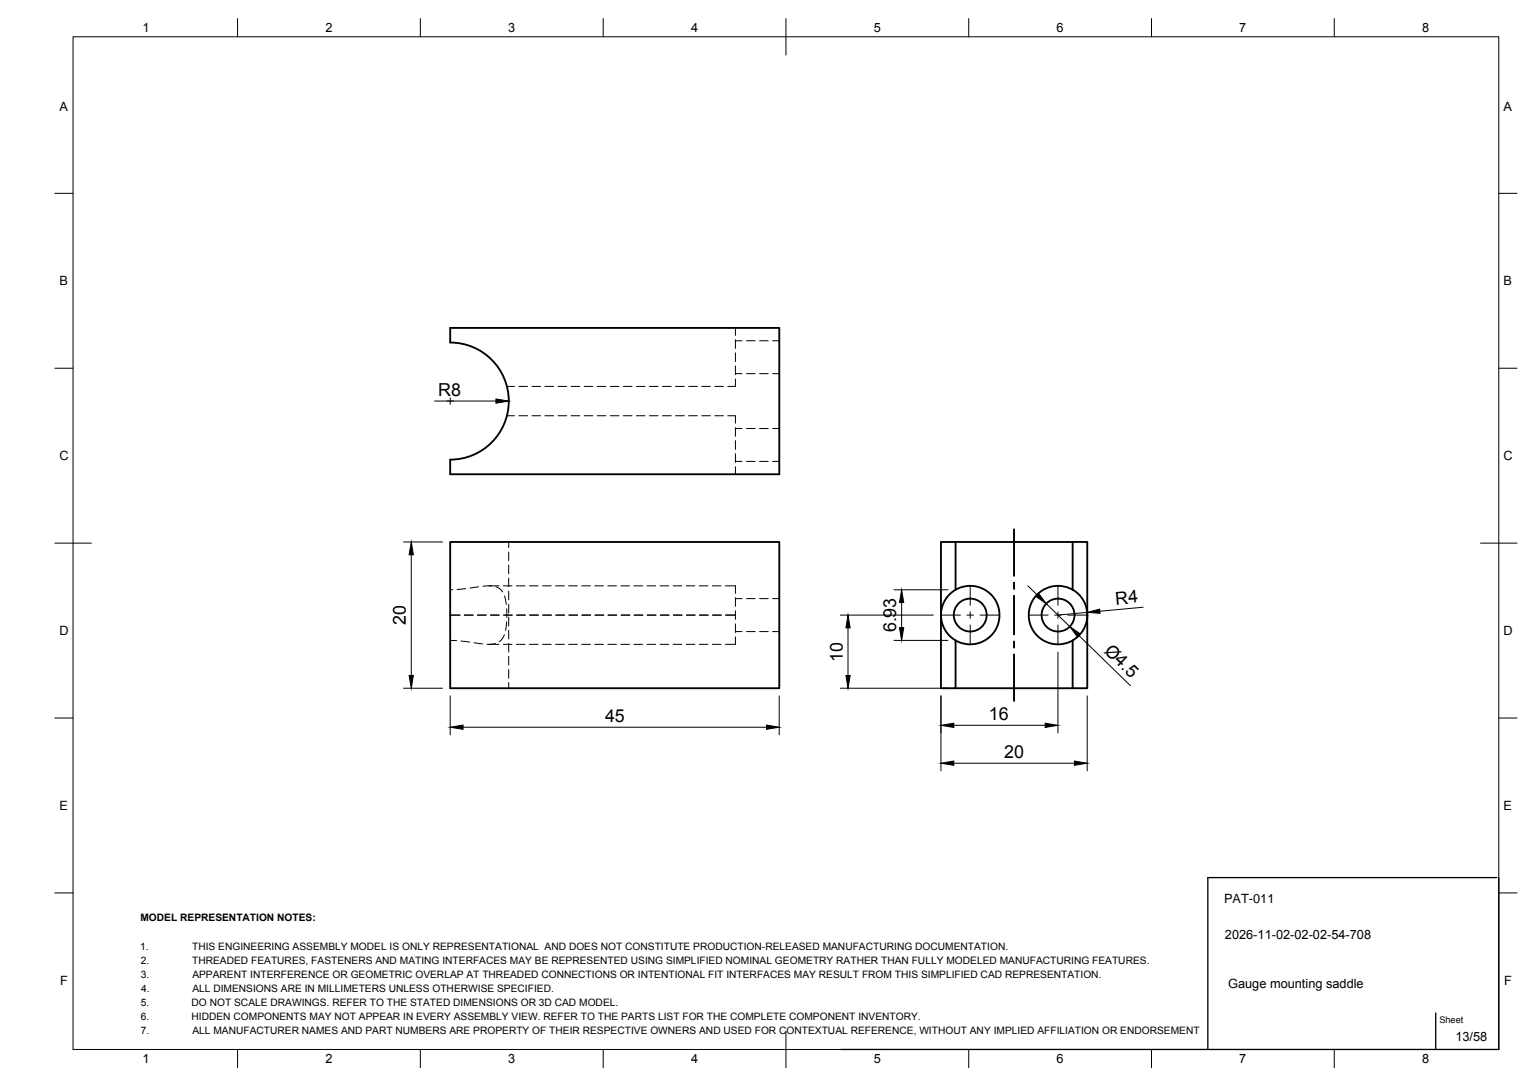
ISO-10303-21;
HEADER;
/* Generated by software containing ST-Developer
 * from STEP Tools, Inc. (www.steptools.com) 
 */

FILE_DESCRIPTION(
/* description */ ('Belt tension measurement rig'),
/* implementation_level */ '2;1');

FILE_NAME(
/* name */ 'Gauge mounting saddle.step',
/* time_stamp */ '2026-10-28T03:24:44-07:00',
/* author */ (''),
/* organization */ (''),
/* preprocessor_version */ 'ST-DEVELOPER v20.2',
/* originating_system */ 'Autodesk Translation Framework v15.17.0.0',
/* authorisation */ '');

FILE_SCHEMA (('AUTOMOTIVE_DESIGN { 1 0 10303 214 3 1 1 }'));
ENDSEC;

DATA;
#10=MECHANICAL_DESIGN_GEOMETRIC_PRESENTATION_REPRESENTATION('',(#704),#23587);
#491=B_SPLINE_CURVE_WITH_KNOTS('',3,(#19153,#19154,#19155,#19156,#19157,
#19158),.UNSPECIFIED.,.F.,.F.,(4,2,4),(1.88587037555333,2.15501811419061,
2.44576925996922),.UNSPECIFIED.);
#492=B_SPLINE_CURVE_WITH_KNOTS('',3,(#19169,#19170,#19171,#19172,#19173,
#19174,#19175,#19176,#19177,#19178,#19179,#19180,#19181,#19182,#19183,#19184,
#19185,#19186,#19187,#19188,#19189,#19190,#19191,#19192,#19193,#19194,#19195,
#19196,#19197,#19198,#19199,#19200),.UNSPECIFIED.,.F.,.F.,(4,2,2,2,2,2,
2,2,2,2,2,2,2,2,2,4),(0.559898884415891,0.581502291557221,0.697930042244281,
0.814357792931341,0.918959320915763,1.02356084890019,1.1232227394424,1.22288462998461,
1.32254652052682,1.42220841106903,1.52680993905346,1.63141146703788,1.74783921772494,
1.864266968412,2.15501811419061,2.44576925996922),.UNSPECIFIED.);
#493=B_SPLINE_CURVE_WITH_KNOTS('',3,(#19203,#19204,#19205,#19206,#19207,
#19208),.UNSPECIFIED.,.F.,.F.,(4,2,4),(0.,0.29075114577861,0.559898884415891),
 .UNSPECIFIED.);
#494=B_SPLINE_CURVE_WITH_KNOTS('',3,(#19217,#19218,#19219,#19220,#19221,
#19222,#19223,#19224,#19225,#19226,#19227,#19228,#19229,#19230,#19231,#19232,
#19233,#19234,#19235,#19236,#19237,#19238,#19239,#19240,#19241,#19242,#19243,
#19244,#19245,#19246,#19247,#19248),.UNSPECIFIED.,.F.,.F.,(4,2,2,2,2,2,
2,2,2,2,2,2,2,2,2,4),(0.,0.29075114577861,0.58150229155722,0.69793004224428,
0.814357792931341,0.918959320915763,1.02356084890019,1.1232227394424,1.22288462998461,
1.32254652052682,1.42220841106904,1.52680993905346,1.63141146703788,1.74783921772494,
1.864266968412,1.88587037555333),.UNSPECIFIED.);
#594=SHAPE_REPRESENTATION_RELATIONSHIP('SRR','None',#23839,#649);
#649=ADVANCED_BREP_SHAPE_REPRESENTATION('',(#774),#23537);
#704=STYLED_ITEM('',(#24197),#774);
#774=MANIFOLD_SOLID_BREP('Body1',#12209);
#891=FACE_BOUND('',#2255,.T.);
#892=FACE_BOUND('',#2258,.T.);
#893=FACE_BOUND('',#2271,.T.);
#894=FACE_BOUND('',#2272,.T.);
#1109=PLANE('',#13155);
#1110=PLANE('',#13160);
#1111=PLANE('',#13162);
#1112=PLANE('',#13163);
#1113=PLANE('',#13164);
#1114=PLANE('',#13172);
#1115=PLANE('',#13173);
#1116=PLANE('',#13174);
#1117=PLANE('',#13175);
#1118=PLANE('',#13176);
#1119=PLANE('',#13177);
#1485=FACE_OUTER_BOUND('',#2251,.T.);
#1486=FACE_OUTER_BOUND('',#2252,.T.);
#1487=FACE_OUTER_BOUND('',#2253,.T.);
#1488=FACE_OUTER_BOUND('',#2254,.T.);
#1489=FACE_OUTER_BOUND('',#2256,.T.);
#1490=FACE_OUTER_BOUND('',#2257,.T.);
#1491=FACE_OUTER_BOUND('',#2259,.T.);
#1492=FACE_OUTER_BOUND('',#2260,.T.);
#1493=FACE_OUTER_BOUND('',#2261,.T.);
#1494=FACE_OUTER_BOUND('',#2262,.T.);
#1495=FACE_OUTER_BOUND('',#2263,.T.);
#1496=FACE_OUTER_BOUND('',#2264,.T.);
#1497=FACE_OUTER_BOUND('',#2265,.T.);
#1498=FACE_OUTER_BOUND('',#2266,.T.);
#1499=FACE_OUTER_BOUND('',#2267,.T.);
#1500=FACE_OUTER_BOUND('',#2268,.T.);
#1501=FACE_OUTER_BOUND('',#2269,.T.);
#1502=FACE_OUTER_BOUND('',#2270,.T.);
#2251=EDGE_LOOP('',(#8472,#8473,#8474,#8475,#8476));
#2252=EDGE_LOOP('',(#8477,#8478,#8479,#8480,#8481));
#2253=EDGE_LOOP('',(#8482,#8483,#8484,#8485,#8486));
#2254=EDGE_LOOP('',(#8487,#8488));
#2255=EDGE_LOOP('',(#8489));
#2256=EDGE_LOOP('',(#8490,#8491,#8492,#8493,#8494));
#2257=EDGE_LOOP('',(#8495,#8496));
#2258=EDGE_LOOP('',(#8497));
#2259=EDGE_LOOP('',(#8498,#8499,#8500,#8501));
#2260=EDGE_LOOP('',(#8502,#8503,#8504,#8505));
#2261=EDGE_LOOP('',(#8506,#8507,#8508,#8509));
#2262=EDGE_LOOP('',(#8510,#8511,#8512,#8513));
#2263=EDGE_LOOP('',(#8514,#8515,#8516,#8517));
#2264=EDGE_LOOP('',(#8518,#8519,#8520,#8521,#8522,#8523,#8524,#8525,#8526,
#8527));
#2265=EDGE_LOOP('',(#8528,#8529,#8530,#8531,#8532,#8533));
#2266=EDGE_LOOP('',(#8534,#8535,#8536,#8537));
#2267=EDGE_LOOP('',(#8538,#8539,#8540,#8541,#8542,#8543,#8544));
#2268=EDGE_LOOP('',(#8545,#8546,#8547,#8548,#8549,#8550,#8551));
#2269=EDGE_LOOP('',(#8552,#8553,#8554,#8555,#8556,#8557));
#2270=EDGE_LOOP('',(#8558,#8559,#8560,#8561));
#2271=EDGE_LOOP('',(#8562));
#2272=EDGE_LOOP('',(#8563));
#3113=LINE('',#19146,#3864);
#3114=LINE('',#19150,#3865);
#3115=LINE('',#19162,#3866);
#3116=LINE('',#19166,#3867);
#3117=LINE('',#19210,#3868);
#3118=LINE('',#19250,#3869);
#3119=LINE('',#19257,#3870);
#3120=LINE('',#19259,#3871);
#3121=LINE('',#19260,#3872);
#3122=LINE('',#19263,#3873);
#3123=LINE('',#19265,#3874);
#3124=LINE('',#19266,#3875);
#3125=LINE('',#19269,#3876);
#3126=LINE('',#19271,#3877);
#3127=LINE('',#19272,#3878);
#3128=LINE('',#19276,#3879);
#3129=LINE('',#19280,#3880);
#3130=LINE('',#19283,#3881);
#3131=LINE('',#19288,#3882);
#3132=LINE('',#19290,#3883);
#3133=LINE('',#19292,#3884);
#3134=LINE('',#19293,#3885);
#3135=LINE('',#19295,#3886);
#3136=LINE('',#19298,#3887);
#3137=LINE('',#19299,#3888);
#3138=LINE('',#19302,#3889);
#3139=LINE('',#19303,#3890);
#3140=LINE('',#19305,#3891);
#3864=VECTOR('',#15204,0.4);
#3865=VECTOR('',#15207,1.);
#3866=VECTOR('',#15212,0.4);
#3867=VECTOR('',#15215,1.);
#3868=VECTOR('',#15222,1.);
#3869=VECTOR('',#15233,1.);
#3870=VECTOR('',#15242,1.);
#3871=VECTOR('',#15243,1.);
#3872=VECTOR('',#15244,1.);
#3873=VECTOR('',#15247,1.);
#3874=VECTOR('',#15248,1.);
#3875=VECTOR('',#15249,1.);
#3876=VECTOR('',#15252,1.);
#3877=VECTOR('',#15253,1.);
#3878=VECTOR('',#15254,1.);
#3879=VECTOR('',#15259,0.225);
#3880=VECTOR('',#15264,0.225);
#3881=VECTOR('',#15267,1.);
#3882=VECTOR('',#15274,1.);
#3883=VECTOR('',#15275,1.);
#3884=VECTOR('',#15276,1.);
#3885=VECTOR('',#15277,1.);
#3886=VECTOR('',#15280,1.);
#3887=VECTOR('',#15283,1.);
#3888=VECTOR('',#15284,1.);
#3889=VECTOR('',#15287,1.);
#3890=VECTOR('',#15288,1.);
#3891=VECTOR('',#15291,1.);
#4592=CIRCLE('',#13147,0.4);
#4593=CIRCLE('',#13148,0.4);
#4594=CIRCLE('',#13150,0.4);
#4595=CIRCLE('',#13151,0.4);
#4596=CIRCLE('',#13153,0.4);
#4597=CIRCLE('',#13154,0.4);
#4598=CIRCLE('',#13156,0.225);
#4599=CIRCLE('',#13158,0.4);
#4600=CIRCLE('',#13159,0.4);
#4601=CIRCLE('',#13161,0.225);
#4602=CIRCLE('',#13166,0.225);
#4603=CIRCLE('',#13168,0.225);
#4604=CIRCLE('',#13170,0.8);
#4605=CIRCLE('',#13171,0.8);
#5416=VERTEX_POINT('',#19144);
#5417=VERTEX_POINT('',#19145);
#5418=VERTEX_POINT('',#19147);
#5419=VERTEX_POINT('',#19149);
#5420=VERTEX_POINT('',#19151);
#5421=VERTEX_POINT('',#19160);
#5422=VERTEX_POINT('',#19161);
#5423=VERTEX_POINT('',#19163);
#5424=VERTEX_POINT('',#19165);
#5425=VERTEX_POINT('',#19167);
#5426=VERTEX_POINT('',#19202);
#5427=VERTEX_POINT('',#19213);
#5428=VERTEX_POINT('',#19216);
#5429=VERTEX_POINT('',#19253);
#5430=VERTEX_POINT('',#19256);
#5431=VERTEX_POINT('',#19258);
#5432=VERTEX_POINT('',#19262);
#5433=VERTEX_POINT('',#19264);
#5434=VERTEX_POINT('',#19268);
#5435=VERTEX_POINT('',#19270);
#5436=VERTEX_POINT('',#19274);
#5437=VERTEX_POINT('',#19278);
#5438=VERTEX_POINT('',#19282);
#5439=VERTEX_POINT('',#19287);
#5440=VERTEX_POINT('',#19289);
#5441=VERTEX_POINT('',#19291);
#5442=VERTEX_POINT('',#19297);
#5443=VERTEX_POINT('',#19301);
#6595=EDGE_CURVE('',#5416,#5417,#3113,.T.);
#6596=EDGE_CURVE('',#5418,#5416,#4592,.T.);
#6597=EDGE_CURVE('',#5418,#5419,#3114,.T.);
#6598=EDGE_CURVE('',#5420,#5419,#4593,.T.);
#6599=EDGE_CURVE('',#5417,#5420,#491,.T.);
#6600=EDGE_CURVE('',#5421,#5422,#3115,.T.);
#6601=EDGE_CURVE('',#5423,#5421,#4594,.T.);
#6602=EDGE_CURVE('',#5423,#5424,#3116,.T.);
#6603=EDGE_CURVE('',#5425,#5424,#4595,.T.);
#6604=EDGE_CURVE('',#5422,#5425,#492,.T.);
#6605=EDGE_CURVE('',#5426,#5422,#493,.T.);
#6606=EDGE_CURVE('',#5424,#5426,#4596,.T.);
#6607=EDGE_CURVE('',#5423,#5424,#3117,.T.);
#6608=EDGE_CURVE('',#5421,#5423,#4597,.T.);
#6609=EDGE_CURVE('',#5427,#5427,#4598,.T.);
#6610=EDGE_CURVE('',#5428,#5417,#494,.T.);
#6611=EDGE_CURVE('',#5419,#5428,#4599,.T.);
#6612=EDGE_CURVE('',#5418,#5419,#3118,.T.);
#6613=EDGE_CURVE('',#5416,#5418,#4600,.T.);
#6614=EDGE_CURVE('',#5429,#5429,#4601,.T.);
#6615=EDGE_CURVE('',#5426,#5430,#3119,.T.);
#6616=EDGE_CURVE('',#5430,#5431,#3120,.T.);
#6617=EDGE_CURVE('',#5431,#5424,#3121,.T.);
#6618=EDGE_CURVE('',#5428,#5432,#3122,.T.);
#6619=EDGE_CURVE('',#5432,#5433,#3123,.T.);
#6620=EDGE_CURVE('',#5433,#5419,#3124,.T.);
#6621=EDGE_CURVE('',#5419,#5434,#3125,.T.);
#6622=EDGE_CURVE('',#5434,#5435,#3126,.T.);
#6623=EDGE_CURVE('',#5435,#5420,#3127,.T.);
#6624=EDGE_CURVE('',#5436,#5436,#4602,.T.);
#6625=EDGE_CURVE('',#5436,#5427,#3128,.T.);
#6626=EDGE_CURVE('',#5437,#5437,#4603,.T.);
#6627=EDGE_CURVE('',#5437,#5429,#3129,.T.);
#6628=EDGE_CURVE('',#5438,#5425,#3130,.T.);
#6629=EDGE_CURVE('',#5432,#5438,#4604,.T.);
#6630=EDGE_CURVE('',#5430,#5435,#4605,.T.);
#6631=EDGE_CURVE('',#5439,#5438,#3131,.T.);
#6632=EDGE_CURVE('',#5440,#5439,#3132,.T.);
#6633=EDGE_CURVE('',#5440,#5441,#3133,.T.);
#6634=EDGE_CURVE('',#5441,#5433,#3134,.T.);
#6635=EDGE_CURVE('',#5424,#5439,#3135,.T.);
#6636=EDGE_CURVE('',#5441,#5442,#3136,.T.);
#6637=EDGE_CURVE('',#5442,#5434,#3137,.T.);
#6638=EDGE_CURVE('',#5443,#5440,#3138,.T.);
#6639=EDGE_CURVE('',#5443,#5431,#3139,.T.);
#6640=EDGE_CURVE('',#5442,#5443,#3140,.T.);
#8472=ORIENTED_EDGE('',*,*,#6595,.F.);
#8473=ORIENTED_EDGE('',*,*,#6596,.F.);
#8474=ORIENTED_EDGE('',*,*,#6597,.T.);
#8475=ORIENTED_EDGE('',*,*,#6598,.F.);
#8476=ORIENTED_EDGE('',*,*,#6599,.F.);
#8477=ORIENTED_EDGE('',*,*,#6600,.F.);
#8478=ORIENTED_EDGE('',*,*,#6601,.F.);
#8479=ORIENTED_EDGE('',*,*,#6602,.T.);
#8480=ORIENTED_EDGE('',*,*,#6603,.F.);
#8481=ORIENTED_EDGE('',*,*,#6604,.F.);
#8482=ORIENTED_EDGE('',*,*,#6600,.T.);
#8483=ORIENTED_EDGE('',*,*,#6605,.F.);
#8484=ORIENTED_EDGE('',*,*,#6606,.F.);
#8485=ORIENTED_EDGE('',*,*,#6607,.F.);
#8486=ORIENTED_EDGE('',*,*,#6608,.F.);
#8487=ORIENTED_EDGE('',*,*,#6601,.T.);
#8488=ORIENTED_EDGE('',*,*,#6608,.T.);
#8489=ORIENTED_EDGE('',*,*,#6609,.F.);
#8490=ORIENTED_EDGE('',*,*,#6595,.T.);
#8491=ORIENTED_EDGE('',*,*,#6610,.F.);
#8492=ORIENTED_EDGE('',*,*,#6611,.F.);
#8493=ORIENTED_EDGE('',*,*,#6612,.F.);
#8494=ORIENTED_EDGE('',*,*,#6613,.F.);
#8495=ORIENTED_EDGE('',*,*,#6596,.T.);
#8496=ORIENTED_EDGE('',*,*,#6613,.T.);
#8497=ORIENTED_EDGE('',*,*,#6614,.F.);
#8498=ORIENTED_EDGE('',*,*,#6606,.T.);
#8499=ORIENTED_EDGE('',*,*,#6615,.T.);
#8500=ORIENTED_EDGE('',*,*,#6616,.T.);
#8501=ORIENTED_EDGE('',*,*,#6617,.T.);
#8502=ORIENTED_EDGE('',*,*,#6611,.T.);
#8503=ORIENTED_EDGE('',*,*,#6618,.T.);
#8504=ORIENTED_EDGE('',*,*,#6619,.T.);
#8505=ORIENTED_EDGE('',*,*,#6620,.T.);
#8506=ORIENTED_EDGE('',*,*,#6598,.T.);
#8507=ORIENTED_EDGE('',*,*,#6621,.T.);
#8508=ORIENTED_EDGE('',*,*,#6622,.T.);
#8509=ORIENTED_EDGE('',*,*,#6623,.T.);
#8510=ORIENTED_EDGE('',*,*,#6624,.F.);
#8511=ORIENTED_EDGE('',*,*,#6625,.T.);
#8512=ORIENTED_EDGE('',*,*,#6609,.T.);
#8513=ORIENTED_EDGE('',*,*,#6625,.F.);
#8514=ORIENTED_EDGE('',*,*,#6626,.F.);
#8515=ORIENTED_EDGE('',*,*,#6627,.T.);
#8516=ORIENTED_EDGE('',*,*,#6614,.T.);
#8517=ORIENTED_EDGE('',*,*,#6627,.F.);
#8518=ORIENTED_EDGE('',*,*,#6605,.T.);
#8519=ORIENTED_EDGE('',*,*,#6604,.T.);
#8520=ORIENTED_EDGE('',*,*,#6628,.F.);
#8521=ORIENTED_EDGE('',*,*,#6629,.F.);
#8522=ORIENTED_EDGE('',*,*,#6618,.F.);
#8523=ORIENTED_EDGE('',*,*,#6610,.T.);
#8524=ORIENTED_EDGE('',*,*,#6599,.T.);
#8525=ORIENTED_EDGE('',*,*,#6623,.F.);
#8526=ORIENTED_EDGE('',*,*,#6630,.F.);
#8527=ORIENTED_EDGE('',*,*,#6615,.F.);
#8528=ORIENTED_EDGE('',*,*,#6629,.T.);
#8529=ORIENTED_EDGE('',*,*,#6631,.F.);
#8530=ORIENTED_EDGE('',*,*,#6632,.F.);
#8531=ORIENTED_EDGE('',*,*,#6633,.T.);
#8532=ORIENTED_EDGE('',*,*,#6634,.T.);
#8533=ORIENTED_EDGE('',*,*,#6619,.F.);
#8534=ORIENTED_EDGE('',*,*,#6603,.T.);
#8535=ORIENTED_EDGE('',*,*,#6635,.T.);
#8536=ORIENTED_EDGE('',*,*,#6631,.T.);
#8537=ORIENTED_EDGE('',*,*,#6628,.T.);
#8538=ORIENTED_EDGE('',*,*,#6636,.T.);
#8539=ORIENTED_EDGE('',*,*,#6637,.T.);
#8540=ORIENTED_EDGE('',*,*,#6621,.F.);
#8541=ORIENTED_EDGE('',*,*,#6597,.F.);
#8542=ORIENTED_EDGE('',*,*,#6612,.T.);
#8543=ORIENTED_EDGE('',*,*,#6620,.F.);
#8544=ORIENTED_EDGE('',*,*,#6634,.F.);
#8545=ORIENTED_EDGE('',*,*,#6638,.T.);
#8546=ORIENTED_EDGE('',*,*,#6632,.T.);
#8547=ORIENTED_EDGE('',*,*,#6635,.F.);
#8548=ORIENTED_EDGE('',*,*,#6602,.F.);
#8549=ORIENTED_EDGE('',*,*,#6607,.T.);
#8550=ORIENTED_EDGE('',*,*,#6617,.F.);
#8551=ORIENTED_EDGE('',*,*,#6639,.F.);
#8552=ORIENTED_EDGE('',*,*,#6630,.T.);
#8553=ORIENTED_EDGE('',*,*,#6622,.F.);
#8554=ORIENTED_EDGE('',*,*,#6637,.F.);
#8555=ORIENTED_EDGE('',*,*,#6640,.T.);
#8556=ORIENTED_EDGE('',*,*,#6639,.T.);
#8557=ORIENTED_EDGE('',*,*,#6616,.F.);
#8558=ORIENTED_EDGE('',*,*,#6640,.F.);
#8559=ORIENTED_EDGE('',*,*,#6636,.F.);
#8560=ORIENTED_EDGE('',*,*,#6633,.F.);
#8561=ORIENTED_EDGE('',*,*,#6638,.F.);
#8562=ORIENTED_EDGE('',*,*,#6624,.T.);
#8563=ORIENTED_EDGE('',*,*,#6626,.T.);
#11219=CYLINDRICAL_SURFACE('',#13146,0.4);
#11220=CYLINDRICAL_SURFACE('',#13149,0.4);
#11221=CYLINDRICAL_SURFACE('',#13152,0.4);
#11222=CYLINDRICAL_SURFACE('',#13157,0.4);
#11223=CYLINDRICAL_SURFACE('',#13165,0.225);
#11224=CYLINDRICAL_SURFACE('',#13167,0.225);
#11225=CYLINDRICAL_SURFACE('',#13169,0.8);
#11626=ADVANCED_FACE('',(#1485),#11219,.F.);
#11627=ADVANCED_FACE('',(#1486),#11220,.F.);
#11628=ADVANCED_FACE('',(#1487),#11221,.F.);
#11629=ADVANCED_FACE('',(#1488,#891),#1109,.T.);
#11630=ADVANCED_FACE('',(#1489),#11222,.F.);
#11631=ADVANCED_FACE('',(#1490,#892),#1110,.T.);
#11632=ADVANCED_FACE('',(#1491),#1111,.T.);
#11633=ADVANCED_FACE('',(#1492),#1112,.T.);
#11634=ADVANCED_FACE('',(#1493),#1113,.T.);
#11635=ADVANCED_FACE('',(#1494),#11223,.F.);
#11636=ADVANCED_FACE('',(#1495),#11224,.F.);
#11637=ADVANCED_FACE('',(#1496),#11225,.F.);
#11638=ADVANCED_FACE('',(#1497),#1114,.T.);
#11639=ADVANCED_FACE('',(#1498),#1115,.T.);
#11640=ADVANCED_FACE('',(#1499),#1116,.T.);
#11641=ADVANCED_FACE('',(#1500),#1117,.T.);
#11642=ADVANCED_FACE('',(#1501),#1118,.T.);
#11643=ADVANCED_FACE('',(#1502,#893,#894),#1119,.F.);
#12209=CLOSED_SHELL('',(#11626,#11627,#11628,#11629,#11630,#11631,#11632,
#11633,#11634,#11635,#11636,#11637,#11638,#11639,#11640,#11641,#11642,#11643));
#13145=AXIS2_PLACEMENT_3D('',#19142,#15200,#15201);
#13146=AXIS2_PLACEMENT_3D('',#19143,#15202,#15203);
#13147=AXIS2_PLACEMENT_3D('',#19148,#15205,#15206);
#13148=AXIS2_PLACEMENT_3D('',#19152,#15208,#15209);
#13149=AXIS2_PLACEMENT_3D('',#19159,#15210,#15211);
#13150=AXIS2_PLACEMENT_3D('',#19164,#15213,#15214);
#13151=AXIS2_PLACEMENT_3D('',#19168,#15216,#15217);
#13152=AXIS2_PLACEMENT_3D('',#19201,#15218,#15219);
#13153=AXIS2_PLACEMENT_3D('',#19209,#15220,#15221);
#13154=AXIS2_PLACEMENT_3D('',#19211,#15223,#15224);
#13155=AXIS2_PLACEMENT_3D('',#19212,#15225,#15226);
#13156=AXIS2_PLACEMENT_3D('',#19214,#15227,#15228);
#13157=AXIS2_PLACEMENT_3D('',#19215,#15229,#15230);
#13158=AXIS2_PLACEMENT_3D('',#19249,#15231,#15232);
#13159=AXIS2_PLACEMENT_3D('',#19251,#15234,#15235);
#13160=AXIS2_PLACEMENT_3D('',#19252,#15236,#15237);
#13161=AXIS2_PLACEMENT_3D('',#19254,#15238,#15239);
#13162=AXIS2_PLACEMENT_3D('',#19255,#15240,#15241);
#13163=AXIS2_PLACEMENT_3D('',#19261,#15245,#15246);
#13164=AXIS2_PLACEMENT_3D('',#19267,#15250,#15251);
#13165=AXIS2_PLACEMENT_3D('',#19273,#15255,#15256);
#13166=AXIS2_PLACEMENT_3D('',#19275,#15257,#15258);
#13167=AXIS2_PLACEMENT_3D('',#19277,#15260,#15261);
#13168=AXIS2_PLACEMENT_3D('',#19279,#15262,#15263);
#13169=AXIS2_PLACEMENT_3D('',#19281,#15265,#15266);
#13170=AXIS2_PLACEMENT_3D('',#19284,#15268,#15269);
#13171=AXIS2_PLACEMENT_3D('',#19285,#15270,#15271);
#13172=AXIS2_PLACEMENT_3D('',#19286,#15272,#15273);
#13173=AXIS2_PLACEMENT_3D('',#19294,#15278,#15279);
#13174=AXIS2_PLACEMENT_3D('',#19296,#15281,#15282);
#13175=AXIS2_PLACEMENT_3D('',#19300,#15285,#15286);
#13176=AXIS2_PLACEMENT_3D('',#19304,#15289,#15290);
#13177=AXIS2_PLACEMENT_3D('',#19306,#15292,#15293);
#15200=DIRECTION('axis',(0.,0.,1.));
#15201=DIRECTION('refdir',(1.,0.,0.));
#15202=DIRECTION('center_axis',(0.,0.,1.));
#15203=DIRECTION('ref_axis',(1.,0.,0.));
#15204=DIRECTION('',(0.,0.,1.));
#15205=DIRECTION('center_axis',(0.,0.,1.));
#15206=DIRECTION('ref_axis',(1.,0.,0.));
#15207=DIRECTION('',(0.,0.,1.));
#15208=DIRECTION('center_axis',(0.,0.,-1.));
#15209=DIRECTION('ref_axis',(1.,0.,0.));
#15210=DIRECTION('center_axis',(0.,0.,1.));
#15211=DIRECTION('ref_axis',(1.,0.,0.));
#15212=DIRECTION('',(0.,0.,1.));
#15213=DIRECTION('center_axis',(0.,0.,1.));
#15214=DIRECTION('ref_axis',(1.,0.,0.));
#15215=DIRECTION('',(0.,0.,1.));
#15216=DIRECTION('center_axis',(0.,0.,-1.));
#15217=DIRECTION('ref_axis',(1.,0.,0.));
#15218=DIRECTION('center_axis',(0.,0.,1.));
#15219=DIRECTION('ref_axis',(1.,0.,0.));
#15220=DIRECTION('center_axis',(0.,0.,-1.));
#15221=DIRECTION('ref_axis',(1.,0.,0.));
#15222=DIRECTION('',(0.,0.,1.));
#15223=DIRECTION('center_axis',(0.,0.,1.));
#15224=DIRECTION('ref_axis',(1.,0.,0.));
#15225=DIRECTION('center_axis',(0.,0.,1.));
#15226=DIRECTION('ref_axis',(1.,0.,0.));
#15227=DIRECTION('center_axis',(0.,0.,1.));
#15228=DIRECTION('ref_axis',(1.,0.,0.));
#15229=DIRECTION('center_axis',(0.,0.,1.));
#15230=DIRECTION('ref_axis',(1.,0.,0.));
#15231=DIRECTION('center_axis',(0.,0.,-1.));
#15232=DIRECTION('ref_axis',(1.,0.,0.));
#15233=DIRECTION('',(0.,0.,1.));
#15234=DIRECTION('center_axis',(0.,0.,1.));
#15235=DIRECTION('ref_axis',(1.,0.,0.));
#15236=DIRECTION('center_axis',(0.,0.,1.));
#15237=DIRECTION('ref_axis',(1.,0.,0.));
#15238=DIRECTION('center_axis',(0.,0.,1.));
#15239=DIRECTION('ref_axis',(1.,0.,0.));
#15240=DIRECTION('center_axis',(0.,0.,1.));
#15241=DIRECTION('ref_axis',(1.,0.,0.));
#15242=DIRECTION('',(-1.,0.,0.));
#15243=DIRECTION('',(0.,-1.,0.));
#15244=DIRECTION('',(1.,0.,0.));
#15245=DIRECTION('center_axis',(0.,0.,1.));
#15246=DIRECTION('ref_axis',(1.,0.,0.));
#15247=DIRECTION('',(1.,0.,0.));
#15248=DIRECTION('',(0.,1.,0.));
#15249=DIRECTION('',(-1.,0.,0.));
#15250=DIRECTION('center_axis',(0.,0.,1.));
#15251=DIRECTION('ref_axis',(1.,0.,0.));
#15252=DIRECTION('',(-1.,0.,0.));
#15253=DIRECTION('',(0.,-1.,0.));
#15254=DIRECTION('',(1.,0.,0.));
#15255=DIRECTION('center_axis',(0.,0.,1.));
#15256=DIRECTION('ref_axis',(1.,0.,0.));
#15257=DIRECTION('center_axis',(0.,0.,1.));
#15258=DIRECTION('ref_axis',(1.,0.,0.));
#15259=DIRECTION('',(0.,0.,1.));
#15260=DIRECTION('center_axis',(0.,0.,1.));
#15261=DIRECTION('ref_axis',(1.,0.,0.));
#15262=DIRECTION('center_axis',(0.,0.,1.));
#15263=DIRECTION('ref_axis',(1.,0.,0.));
#15264=DIRECTION('',(0.,0.,1.));
#15265=DIRECTION('center_axis',(1.,0.,0.));
#15266=DIRECTION('ref_axis',(0.,0.,-1.));
#15267=DIRECTION('',(-1.,0.,0.));
#15268=DIRECTION('center_axis',(-1.,0.,0.));
#15269=DIRECTION('ref_axis',(0.,0.,-1.));
#15270=DIRECTION('center_axis',(1.,0.,0.));
#15271=DIRECTION('ref_axis',(0.,0.,-1.));
#15272=DIRECTION('center_axis',(1.,0.,0.));
#15273=DIRECTION('ref_axis',(0.,1.,0.));
#15274=DIRECTION('',(0.,1.,0.));
#15275=DIRECTION('',(0.,0.,1.));
#15276=DIRECTION('',(0.,1.,0.));
#15277=DIRECTION('',(0.,0.,1.));
#15278=DIRECTION('center_axis',(0.,0.,1.));
#15279=DIRECTION('ref_axis',(1.,0.,0.));
#15280=DIRECTION('',(1.,0.,0.));
#15281=DIRECTION('center_axis',(0.,1.,0.));
#15282=DIRECTION('ref_axis',(-1.,0.,0.));
#15283=DIRECTION('',(-1.,0.,0.));
#15284=DIRECTION('',(0.,0.,1.));
#15285=DIRECTION('center_axis',(0.,-1.,0.));
#15286=DIRECTION('ref_axis',(1.,0.,0.));
#15287=DIRECTION('',(1.,0.,0.));
#15288=DIRECTION('',(0.,0.,1.));
#15289=DIRECTION('center_axis',(-1.,0.,0.));
#15290=DIRECTION('ref_axis',(0.,-1.,0.));
#15291=DIRECTION('',(0.,-1.,0.));
#15292=DIRECTION('center_axis',(0.,0.,1.));
#15293=DIRECTION('ref_axis',(1.,0.,0.));
#19142=CARTESIAN_POINT('',(0.,0.,0.));
#19143=CARTESIAN_POINT('Origin',(3.,8.1,0.6));
#19144=CARTESIAN_POINT('',(2.6,8.1,0.6));
#19145=CARTESIAN_POINT('',(2.6,8.09999999996984,3.97084973771869));
#19146=CARTESIAN_POINT('',(2.6,8.1,0.6));
#19147=CARTESIAN_POINT('',(3.,8.5,0.6));
#19148=CARTESIAN_POINT('Origin',(3.,8.1,0.6));
#19149=CARTESIAN_POINT('',(3.,8.5,4.5));
#19150=CARTESIAN_POINT('',(3.,8.5,0.6));
#19151=CARTESIAN_POINT('',(2.65358983848623,8.3,4.5));
#19152=CARTESIAN_POINT('Origin',(3.,8.1,4.5));
#19153=CARTESIAN_POINT('Ctrl Pts',(2.6,8.09999999993968,3.97084973771869));
#19154=CARTESIAN_POINT('Ctrl Pts',(2.59999999999099,8.15972702790978,4.0385738216565));
#19155=CARTESIAN_POINT('Ctrl Pts',(2.61364657269785,8.209952841357,4.11951904386589));
#19156=CARTESIAN_POINT('Ctrl Pts',(2.64131535047873,8.28146961928914,4.3010711770996));
#19157=CARTESIAN_POINT('Ctrl Pts',(2.65358983848622,8.3,4.40308295140713));
#19158=CARTESIAN_POINT('Ctrl Pts',(2.65358983848622,8.3,4.5));
#19159=CARTESIAN_POINT('Origin',(3.,6.9,0.6));
#19160=CARTESIAN_POINT('',(2.6,6.9,0.6));
#19161=CARTESIAN_POINT('',(2.6,6.90000000003016,3.97084973771869));
#19162=CARTESIAN_POINT('',(2.6,6.9,0.6));
#19163=CARTESIAN_POINT('',(3.,6.5,0.6));
#19164=CARTESIAN_POINT('Origin',(3.,6.9,0.6));
#19165=CARTESIAN_POINT('',(3.,6.5,4.5));
#19166=CARTESIAN_POINT('',(3.,6.5,0.6));
#19167=CARTESIAN_POINT('',(3.34641016151378,6.7,4.5));
#19168=CARTESIAN_POINT('Origin',(3.,6.9,4.5));
#19169=CARTESIAN_POINT('Ctrl Pts',(2.6,6.90000000006032,3.97084973771869));
#19170=CARTESIAN_POINT('Ctrl Pts',(2.60000000000072,6.90479404852274,3.96541379771789));
#19171=CARTESIAN_POINT('Ctrl Pts',(2.60008620085532,6.90964651743076,3.96006056814498));
#19172=CARTESIAN_POINT('Ctrl Pts',(2.60122740656895,6.94099338970816,3.92640010376094));
#19173=CARTESIAN_POINT('Ctrl Pts',(2.60512454705338,6.97203740815281,3.89755171629685));
#19174=CARTESIAN_POINT('Ctrl Pts',(2.6225443141011,7.03654018405112,3.8466291847403));
#19175=CARTESIAN_POINT('Ctrl Pts',(2.63623381415265,7.06993848403684,3.82453570130603));
#19176=CARTESIAN_POINT('Ctrl Pts',(2.66918291362779,7.12700799839143,3.79158660183088));
#19177=CARTESIAN_POINT('Ctrl Pts',(2.69015083258595,7.15550942144409,3.77743263176733));
#19178=CARTESIAN_POINT('Ctrl Pts',(2.74065869020899,7.20664909771142,3.75520298086526));
#19179=CARTESIAN_POINT('Ctrl Pts',(2.77021713882404,7.2292150185966,3.74700319058552));
#19180=CARTESIAN_POINT('Ctrl Pts',(2.82837641387987,7.26279329170595,3.73578055053196));
#19181=CARTESIAN_POINT('Ctrl Pts',(2.8615419983492,7.27697903270593,3.73165447370246));
#19182=CARTESIAN_POINT('Ctrl Pts',(2.93074503613534,7.29558509017111,3.72649645101547));
#19183=CARTESIAN_POINT('Ctrl Pts',(2.96677936981926,7.3,3.72540333075852));
#19184=CARTESIAN_POINT('Ctrl Pts',(3.03322063018074,7.3,3.72540333075852));
#19185=CARTESIAN_POINT('Ctrl Pts',(3.06925496386466,7.29558509017111,3.72649645101547));
#19186=CARTESIAN_POINT('Ctrl Pts',(3.1384580016508,7.27697903270593,3.73165447370246));
#19187=CARTESIAN_POINT('Ctrl Pts',(3.17162358612013,7.26279329170596,3.73578055053196));
#19188=CARTESIAN_POINT('Ctrl Pts',(3.22978286117596,7.2292150185966,3.74700319058552));
#19189=CARTESIAN_POINT('Ctrl Pts',(3.25934130979101,7.20664909771142,3.75520298086526));
#19190=CARTESIAN_POINT('Ctrl Pts',(3.30984916741405,7.15550942144409,3.77743263176733));
#19191=CARTESIAN_POINT('Ctrl Pts',(3.33081708637221,7.12700799839143,3.79158660183088));
#19192=CARTESIAN_POINT('Ctrl Pts',(3.36376618584735,7.06993848403684,3.82453570130603));
#19193=CARTESIAN_POINT('Ctrl Pts',(3.3774556858989,7.03654018405112,3.8466291847403));
#19194=CARTESIAN_POINT('Ctrl Pts',(3.39487545294662,6.97203740815281,3.89755171629685));
#19195=CARTESIAN_POINT('Ctrl Pts',(3.39877259343105,6.94099338970816,3.92640010376094));
#19196=CARTESIAN_POINT('Ctrl Pts',(3.40213904264749,6.84852307313348,4.02569529883171));
#19197=CARTESIAN_POINT('Ctrl Pts',(3.38742101269684,6.79280659630953,4.11251394926614));
#19198=CARTESIAN_POINT('Ctrl Pts',(3.35868464952127,6.71853038071086,4.3010711770996));
#19199=CARTESIAN_POINT('Ctrl Pts',(3.34641016151378,6.7,4.40308295140713));
#19200=CARTESIAN_POINT('Ctrl Pts',(3.34641016151378,6.7,4.5));
#19201=CARTESIAN_POINT('Origin',(3.,6.9,0.6));
#19202=CARTESIAN_POINT('',(2.65358983848622,6.7,4.5));
#19203=CARTESIAN_POINT('Ctrl Pts',(2.65358983848622,6.7,4.5));
#19204=CARTESIAN_POINT('Ctrl Pts',(2.65358983848622,6.7,4.40308295140713));
#19205=CARTESIAN_POINT('Ctrl Pts',(2.64131535047873,6.71853038071086,4.3010711770996));
#19206=CARTESIAN_POINT('Ctrl Pts',(2.61364657269785,6.790047158643,4.11951904386589));
#19207=CARTESIAN_POINT('Ctrl Pts',(2.59999999999099,6.84027297209022,4.0385738216565));
#19208=CARTESIAN_POINT('Ctrl Pts',(2.6,6.90000000006032,3.97084973771869));
#19209=CARTESIAN_POINT('Origin',(3.,6.9,4.5));
#19210=CARTESIAN_POINT('',(3.,6.5,0.6));
#19211=CARTESIAN_POINT('Origin',(3.,6.9,0.6));
#19212=CARTESIAN_POINT('Origin',(3.,6.9,0.6));
#19213=CARTESIAN_POINT('',(2.775,6.9,0.6));
#19214=CARTESIAN_POINT('Origin',(3.,6.9,0.6));
#19215=CARTESIAN_POINT('Origin',(3.,8.1,0.6));
#19216=CARTESIAN_POINT('',(3.34641016151377,8.3,4.5));
#19217=CARTESIAN_POINT('Ctrl Pts',(3.34641016151378,8.3,4.5));
#19218=CARTESIAN_POINT('Ctrl Pts',(3.34641016151378,8.3,4.40308295140713));
#19219=CARTESIAN_POINT('Ctrl Pts',(3.35868464952127,8.28146961928914,4.3010711770996));
#19220=CARTESIAN_POINT('Ctrl Pts',(3.38742101269684,8.20719340369047,4.11251394926615));
#19221=CARTESIAN_POINT('Ctrl Pts',(3.40213904264749,8.15147692686652,4.02569529883171));
#19222=CARTESIAN_POINT('Ctrl Pts',(3.39877259343105,8.05900661029184,3.92640010376094));
#19223=CARTESIAN_POINT('Ctrl Pts',(3.39487545294662,8.02796259184719,3.89755171629685));
#19224=CARTESIAN_POINT('Ctrl Pts',(3.3774556858989,7.96345981594888,3.8466291847403));
#19225=CARTESIAN_POINT('Ctrl Pts',(3.36376618584735,7.93006151596316,3.82453570130603));
#19226=CARTESIAN_POINT('Ctrl Pts',(3.33081708637221,7.87299200160857,3.79158660183088));
#19227=CARTESIAN_POINT('Ctrl Pts',(3.30984916741405,7.84449057855591,3.77743263176733));
#19228=CARTESIAN_POINT('Ctrl Pts',(3.25934130979101,7.79335090228858,3.75520298086526));
#19229=CARTESIAN_POINT('Ctrl Pts',(3.22978286117596,7.7707849814034,3.74700319058552));
#19230=CARTESIAN_POINT('Ctrl Pts',(3.17162358612013,7.73720670829404,3.73578055053196));
#19231=CARTESIAN_POINT('Ctrl Pts',(3.1384580016508,7.72302096729407,3.73165447370246));
#19232=CARTESIAN_POINT('Ctrl Pts',(3.06925496386466,7.70441490982889,3.72649645101547));
#19233=CARTESIAN_POINT('Ctrl Pts',(3.03322063018074,7.7,3.72540333075852));
#19234=CARTESIAN_POINT('Ctrl Pts',(2.96677936981926,7.7,3.72540333075852));
#19235=CARTESIAN_POINT('Ctrl Pts',(2.93074503613534,7.70441490982889,3.72649645101547));
#19236=CARTESIAN_POINT('Ctrl Pts',(2.8615419983492,7.72302096729407,3.73165447370246));
#19237=CARTESIAN_POINT('Ctrl Pts',(2.82837641387987,7.73720670829404,3.73578055053196));
#19238=CARTESIAN_POINT('Ctrl Pts',(2.77021713882404,7.7707849814034,3.74700319058552));
#19239=CARTESIAN_POINT('Ctrl Pts',(2.74065869020899,7.79335090228858,3.75520298086526));
#19240=CARTESIAN_POINT('Ctrl Pts',(2.69015083258595,7.84449057855591,3.77743263176733));
#19241=CARTESIAN_POINT('Ctrl Pts',(2.66918291362779,7.87299200160857,3.79158660183088));
#19242=CARTESIAN_POINT('Ctrl Pts',(2.63623381415265,7.93006151596316,3.82453570130603));
#19243=CARTESIAN_POINT('Ctrl Pts',(2.6225443141011,7.96345981594888,3.8466291847403));
#19244=CARTESIAN_POINT('Ctrl Pts',(2.60512454705338,8.02796259184719,3.89755171629685));
#19245=CARTESIAN_POINT('Ctrl Pts',(2.60122740656895,8.05900661029184,3.92640010376094));
#19246=CARTESIAN_POINT('Ctrl Pts',(2.60008620085532,8.09035348256924,3.96006056814498));
#19247=CARTESIAN_POINT('Ctrl Pts',(2.60000000000072,8.09520595147726,3.96541379771789));
#19248=CARTESIAN_POINT('Ctrl Pts',(2.6,8.09999999993968,3.97084973771869));
#19249=CARTESIAN_POINT('Origin',(3.,8.1,4.5));
#19250=CARTESIAN_POINT('',(3.,8.5,0.6));
#19251=CARTESIAN_POINT('Origin',(3.,8.1,0.6));
#19252=CARTESIAN_POINT('Origin',(3.,8.1,0.6));
#19253=CARTESIAN_POINT('',(2.775,8.1,0.6));
#19254=CARTESIAN_POINT('Origin',(3.,8.1,0.6));
#19255=CARTESIAN_POINT('Origin',(3.,7.5,4.5));
#19256=CARTESIAN_POINT('',(2.,6.7,4.5));
#19257=CARTESIAN_POINT('',(1.9,6.7,4.5));
#19258=CARTESIAN_POINT('',(2.,6.5,4.5));
#19259=CARTESIAN_POINT('',(2.,8.5,4.5));
#19260=CARTESIAN_POINT('',(2.,6.5,4.5));
#19261=CARTESIAN_POINT('Origin',(3.,7.5,4.5));
#19262=CARTESIAN_POINT('',(4.,8.3,4.5));
#19263=CARTESIAN_POINT('',(1.9,8.3,4.5));
#19264=CARTESIAN_POINT('',(4.,8.5,4.5));
#19265=CARTESIAN_POINT('',(4.,6.5,4.5));
#19266=CARTESIAN_POINT('',(4.,8.5,4.5));
#19267=CARTESIAN_POINT('Origin',(3.,7.5,4.5));
#19268=CARTESIAN_POINT('',(2.,8.5,4.5));
#19269=CARTESIAN_POINT('',(4.,8.5,4.5));
#19270=CARTESIAN_POINT('',(2.,8.3,4.5));
#19271=CARTESIAN_POINT('',(2.,8.5,4.5));
#19272=CARTESIAN_POINT('',(1.9,8.3,4.5));
#19273=CARTESIAN_POINT('Origin',(3.,6.9,-0.1));
#19274=CARTESIAN_POINT('',(2.775,6.9,0.));
#19275=CARTESIAN_POINT('Origin',(3.,6.9,0.));
#19276=CARTESIAN_POINT('',(2.775,6.9,-0.1));
#19277=CARTESIAN_POINT('Origin',(3.,8.1,-0.1));
#19278=CARTESIAN_POINT('',(2.775,8.1,0.));
#19279=CARTESIAN_POINT('Origin',(3.,8.1,0.));
#19280=CARTESIAN_POINT('',(2.775,8.1,-0.1));
#19281=CARTESIAN_POINT('Origin',(1.9,7.5,4.5));
#19282=CARTESIAN_POINT('',(4.,6.7,4.5));
#19283=CARTESIAN_POINT('',(1.9,6.7,4.5));
#19284=CARTESIAN_POINT('Origin',(4.,7.5,4.5));
#19285=CARTESIAN_POINT('Origin',(2.,7.5,4.5));
#19286=CARTESIAN_POINT('Origin',(4.,6.5,0.));
#19287=CARTESIAN_POINT('',(4.,6.5,4.5));
#19288=CARTESIAN_POINT('',(4.,6.5,4.5));
#19289=CARTESIAN_POINT('',(4.,6.5,0.));
#19290=CARTESIAN_POINT('',(4.,6.5,0.));
#19291=CARTESIAN_POINT('',(4.,8.5,0.));
#19292=CARTESIAN_POINT('',(4.,6.5,0.));
#19293=CARTESIAN_POINT('',(4.,8.5,0.));
#19294=CARTESIAN_POINT('Origin',(3.,7.5,4.5));
#19295=CARTESIAN_POINT('',(2.,6.5,4.5));
#19296=CARTESIAN_POINT('Origin',(4.,8.5,0.));
#19297=CARTESIAN_POINT('',(2.,8.5,0.));
#19298=CARTESIAN_POINT('',(4.,8.5,0.));
#19299=CARTESIAN_POINT('',(2.,8.5,0.));
#19300=CARTESIAN_POINT('Origin',(2.,6.5,0.));
#19301=CARTESIAN_POINT('',(2.,6.5,0.));
#19302=CARTESIAN_POINT('',(2.,6.5,0.));
#19303=CARTESIAN_POINT('',(2.,6.5,0.));
#19304=CARTESIAN_POINT('Origin',(2.,8.5,0.));
#19305=CARTESIAN_POINT('',(2.,8.5,0.));
#19306=CARTESIAN_POINT('Origin',(3.,7.5,0.));
#23472=UNCERTAINTY_MEASURE_WITH_UNIT(LENGTH_MEASURE(0.001),#23588,
'DISTANCE_ACCURACY_VALUE',
'Maximum model space distance between geometric entities at asserted c
onnectivities');
#23522=UNCERTAINTY_MEASURE_WITH_UNIT(LENGTH_MEASURE(0.001),#23588,
'DISTANCE_ACCURACY_VALUE',
'Maximum model space distance between geometric entities at asserted c
onnectivities');
#23537=(
GEOMETRIC_REPRESENTATION_CONTEXT(3)
GLOBAL_UNCERTAINTY_ASSIGNED_CONTEXT((#23472))
GLOBAL_UNIT_ASSIGNED_CONTEXT((#23588,#23590,#23591))
REPRESENTATION_CONTEXT('','3D')
);
#23587=(
GEOMETRIC_REPRESENTATION_CONTEXT(3)
GLOBAL_UNCERTAINTY_ASSIGNED_CONTEXT((#23522))
GLOBAL_UNIT_ASSIGNED_CONTEXT((#23588,#23590,#23591))
REPRESENTATION_CONTEXT('','3D')
);
#23588=(
LENGTH_UNIT()
NAMED_UNIT(*)
SI_UNIT(.CENTI.,.METRE.)
);
#23590=(
NAMED_UNIT(*)
PLANE_ANGLE_UNIT()
SI_UNIT($,.RADIAN.)
);
#23591=(
NAMED_UNIT(*)
SI_UNIT($,.STERADIAN.)
SOLID_ANGLE_UNIT()
);
#23606=SHAPE_DEFINITION_REPRESENTATION(#23670,#23839);
#23670=PRODUCT_DEFINITION_SHAPE('',$,#23904);
#23839=SHAPE_REPRESENTATION('',(#13145),#23537);
#23889=PRODUCT_DEFINITION_CONTEXT('part definition',#24083,'design');
#23904=PRODUCT_DEFINITION('Gauge mounting saddle',
'Gauge mounting saddle',#23968,#23889);
#23968=PRODUCT_DEFINITION_FORMATION('',$,#24099);
#24083=APPLICATION_CONTEXT(
'Core Data for Automotive Mechanical Design Process');
#24084=PRODUCT_CONTEXT('part definition',#24083,'mechanical');
#24099=PRODUCT('Gauge mounting saddle','Gauge mounting saddle',
'Gauge mounting saddle',(#24084));
#24191=COLOUR_RGB('Light Blue',0.38,0.62,0.78);
#24192=FILL_AREA_STYLE_COLOUR('',#24191);
#24193=FILL_AREA_STYLE('',(#24192));
#24194=SURFACE_STYLE_FILL_AREA(#24193);
#24195=SURFACE_SIDE_STYLE('',(#24194));
#24196=SURFACE_STYLE_USAGE(.BOTH.,#24195);
#24197=PRESENTATION_STYLE_ASSIGNMENT((#24196));
ENDSEC;
END-ISO-10303-21;
